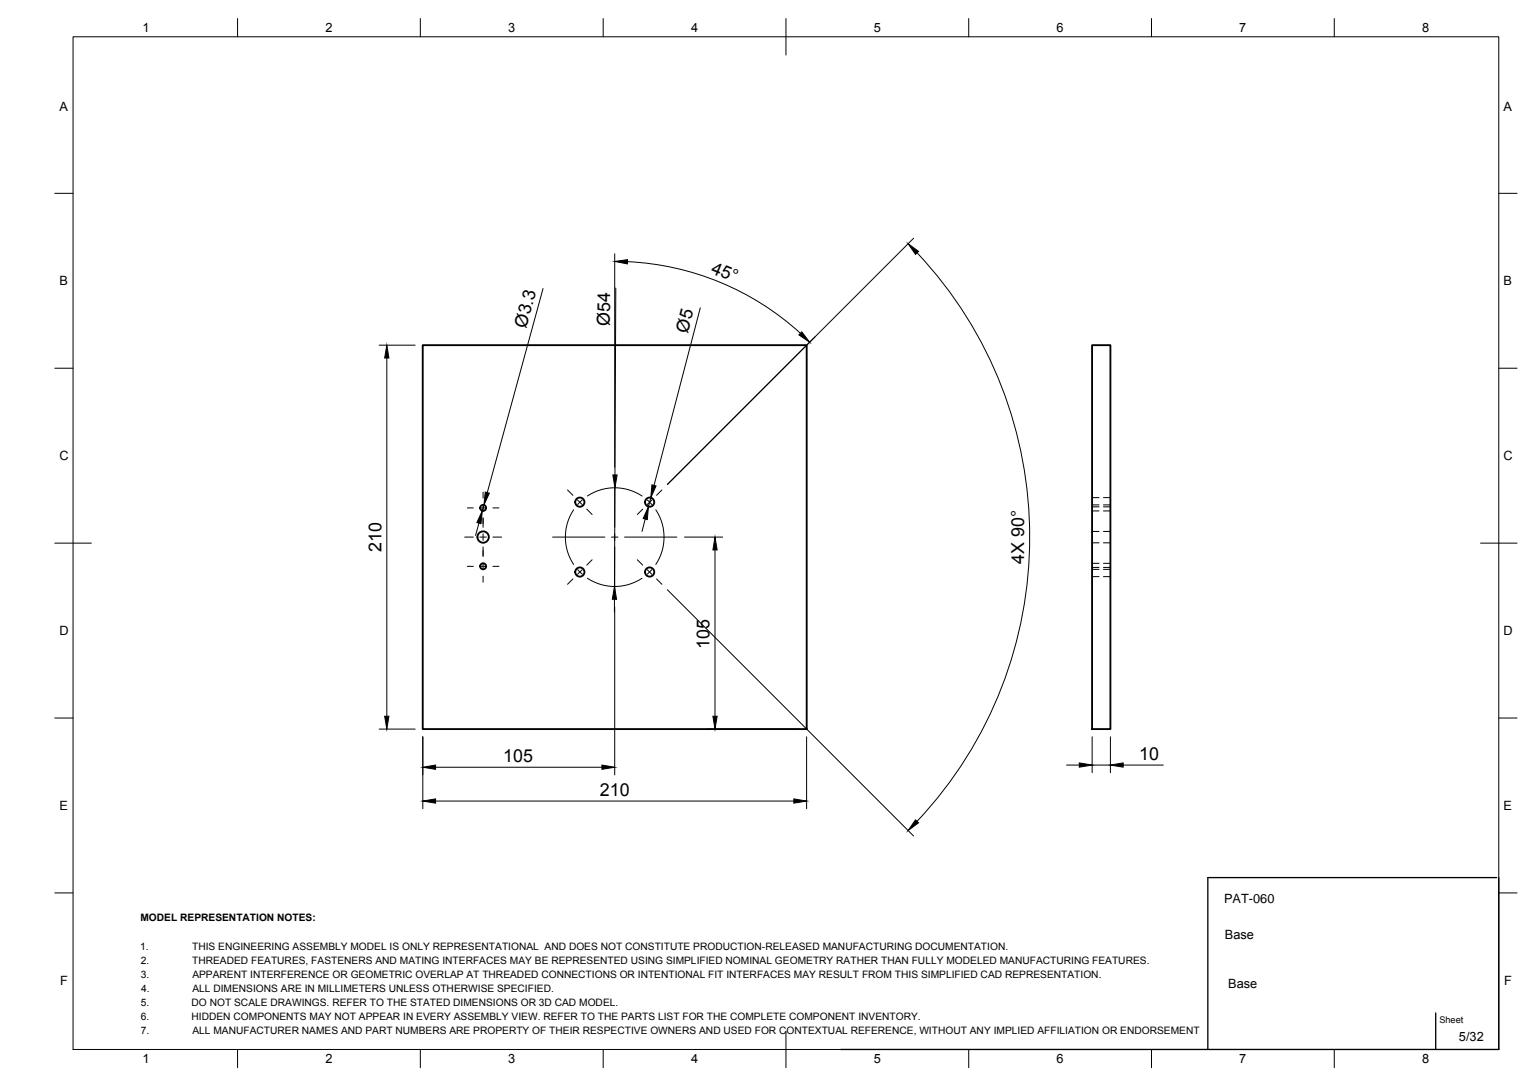
ISO-10303-21;
HEADER;
/* Generated by software containing ST-Developer
 * from STEP Tools, Inc. (www.steptools.com) 
 */

FILE_DESCRIPTION(
/* description */ ('Indexing fixture plate with plunger'),
/* implementation_level */ '2;1');

FILE_NAME(
/* name */ 'Base.step',
/* time_stamp */ '2026-10-28T03:23:41-07:00',
/* author */ (''),
/* organization */ (''),
/* preprocessor_version */ 'ST-DEVELOPER v20.2',
/* originating_system */ 'Autodesk Translation Framework v15.17.0.0',
/* authorisation */ '');

FILE_SCHEMA (('AUTOMOTIVE_DESIGN { 1 0 10303 214 3 1 1 }'));
ENDSEC;

DATA;
#10=MECHANICAL_DESIGN_GEOMETRIC_PRESENTATION_REPRESENTATION('',(#317),#10020);
#263=SHAPE_REPRESENTATION_RELATIONSHIP('SRR','None',#10137,#290);
#290=ADVANCED_BREP_SHAPE_REPRESENTATION('',(#353),#9990);
#317=STYLED_ITEM('',(#10347),#353);
#353=MANIFOLD_SOLID_BREP('Body1',#4571);
#387=FACE_BOUND('',#968,.T.);
#388=FACE_BOUND('',#969,.T.);
#389=FACE_BOUND('',#970,.T.);
#390=FACE_BOUND('',#971,.T.);
#391=FACE_BOUND('',#972,.T.);
#392=FACE_BOUND('',#973,.T.);
#393=FACE_BOUND('',#974,.T.);
#394=FACE_BOUND('',#976,.T.);
#395=FACE_BOUND('',#977,.T.);
#396=FACE_BOUND('',#978,.T.);
#397=FACE_BOUND('',#979,.T.);
#398=FACE_BOUND('',#980,.T.);
#399=FACE_BOUND('',#981,.T.);
#400=FACE_BOUND('',#982,.T.);
#537=PLANE('',#4931);
#538=PLANE('',#4932);
#539=PLANE('',#4933);
#540=PLANE('',#4934);
#541=PLANE('',#4935);
#542=PLANE('',#4936);
#670=FACE_OUTER_BOUND('',#956,.T.);
#671=FACE_OUTER_BOUND('',#957,.T.);
#672=FACE_OUTER_BOUND('',#958,.T.);
#673=FACE_OUTER_BOUND('',#959,.T.);
#674=FACE_OUTER_BOUND('',#960,.T.);
#675=FACE_OUTER_BOUND('',#961,.T.);
#676=FACE_OUTER_BOUND('',#962,.T.);
#677=FACE_OUTER_BOUND('',#963,.T.);
#678=FACE_OUTER_BOUND('',#964,.T.);
#679=FACE_OUTER_BOUND('',#965,.T.);
#680=FACE_OUTER_BOUND('',#966,.T.);
#681=FACE_OUTER_BOUND('',#967,.T.);
#682=FACE_OUTER_BOUND('',#975,.T.);
#956=EDGE_LOOP('',(#3063,#3064,#3065,#3066));
#957=EDGE_LOOP('',(#3067,#3068,#3069,#3070));
#958=EDGE_LOOP('',(#3071,#3072,#3073,#3074));
#959=EDGE_LOOP('',(#3075,#3076,#3077,#3078));
#960=EDGE_LOOP('',(#3079,#3080,#3081,#3082));
#961=EDGE_LOOP('',(#3083,#3084,#3085,#3086));
#962=EDGE_LOOP('',(#3087,#3088,#3089,#3090));
#963=EDGE_LOOP('',(#3091,#3092,#3093,#3094));
#964=EDGE_LOOP('',(#3095,#3096,#3097,#3098));
#965=EDGE_LOOP('',(#3099,#3100,#3101,#3102));
#966=EDGE_LOOP('',(#3103,#3104,#3105,#3106));
#967=EDGE_LOOP('',(#3107,#3108,#3109,#3110));
#968=EDGE_LOOP('',(#3111));
#969=EDGE_LOOP('',(#3112));
#970=EDGE_LOOP('',(#3113));
#971=EDGE_LOOP('',(#3114));
#972=EDGE_LOOP('',(#3115));
#973=EDGE_LOOP('',(#3116));
#974=EDGE_LOOP('',(#3117));
#975=EDGE_LOOP('',(#3118,#3119,#3120,#3121));
#976=EDGE_LOOP('',(#3122));
#977=EDGE_LOOP('',(#3123));
#978=EDGE_LOOP('',(#3124));
#979=EDGE_LOOP('',(#3125));
#980=EDGE_LOOP('',(#3126));
#981=EDGE_LOOP('',(#3127));
#982=EDGE_LOOP('',(#3128));
#1392=LINE('',#7132,#1612);
#1393=LINE('',#7138,#1613);
#1394=LINE('',#7144,#1614);
#1395=LINE('',#7150,#1615);
#1396=LINE('',#7156,#1616);
#1397=LINE('',#7162,#1617);
#1398=LINE('',#7168,#1618);
#1399=LINE('',#7173,#1619);
#1400=LINE('',#7175,#1620);
#1401=LINE('',#7177,#1621);
#1402=LINE('',#7178,#1622);
#1403=LINE('',#7181,#1623);
#1404=LINE('',#7183,#1624);
#1405=LINE('',#7184,#1625);
#1406=LINE('',#7187,#1626);
#1407=LINE('',#7189,#1627);
#1408=LINE('',#7190,#1628);
#1409=LINE('',#7192,#1629);
#1410=LINE('',#7193,#1630);
#1612=VECTOR('',#5583,0.165);
#1613=VECTOR('',#5590,0.165);
#1614=VECTOR('',#5597,0.31);
#1615=VECTOR('',#5604,0.25);
#1616=VECTOR('',#5611,0.25);
#1617=VECTOR('',#5618,0.25);
#1618=VECTOR('',#5625,0.25);
#1619=VECTOR('',#5630,1.);
#1620=VECTOR('',#5631,1.);
#1621=VECTOR('',#5632,1.);
#1622=VECTOR('',#5633,1.);
#1623=VECTOR('',#5636,1.);
#1624=VECTOR('',#5637,1.);
#1625=VECTOR('',#5638,1.);
#1626=VECTOR('',#5641,1.);
#1627=VECTOR('',#5642,1.);
#1628=VECTOR('',#5643,1.);
#1629=VECTOR('',#5646,1.);
#1630=VECTOR('',#5647,1.);
#1832=CIRCLE('',#4911,0.165);
#1833=CIRCLE('',#4912,0.165);
#1834=CIRCLE('',#4914,0.165);
#1835=CIRCLE('',#4915,0.165);
#1836=CIRCLE('',#4917,0.31);
#1837=CIRCLE('',#4918,0.31);
#1838=CIRCLE('',#4920,0.25);
#1839=CIRCLE('',#4921,0.25);
#1840=CIRCLE('',#4923,0.25);
#1841=CIRCLE('',#4924,0.25);
#1842=CIRCLE('',#4926,0.25);
#1843=CIRCLE('',#4927,0.25);
#1844=CIRCLE('',#4929,0.25);
#1845=CIRCLE('',#4930,0.25);
#2135=VERTEX_POINT('',#7129);
#2136=VERTEX_POINT('',#7131);
#2137=VERTEX_POINT('',#7135);
#2138=VERTEX_POINT('',#7137);
#2139=VERTEX_POINT('',#7141);
#2140=VERTEX_POINT('',#7143);
#2141=VERTEX_POINT('',#7147);
#2142=VERTEX_POINT('',#7149);
#2143=VERTEX_POINT('',#7153);
#2144=VERTEX_POINT('',#7155);
#2145=VERTEX_POINT('',#7159);
#2146=VERTEX_POINT('',#7161);
#2147=VERTEX_POINT('',#7165);
#2148=VERTEX_POINT('',#7167);
#2149=VERTEX_POINT('',#7171);
#2150=VERTEX_POINT('',#7172);
#2151=VERTEX_POINT('',#7174);
#2152=VERTEX_POINT('',#7176);
#2153=VERTEX_POINT('',#7180);
#2154=VERTEX_POINT('',#7182);
#2155=VERTEX_POINT('',#7186);
#2156=VERTEX_POINT('',#7188);
#2511=EDGE_CURVE('',#2135,#2135,#1832,.T.);
#2512=EDGE_CURVE('',#2135,#2136,#1392,.T.);
#2513=EDGE_CURVE('',#2136,#2136,#1833,.T.);
#2514=EDGE_CURVE('',#2137,#2137,#1834,.T.);
#2515=EDGE_CURVE('',#2137,#2138,#1393,.T.);
#2516=EDGE_CURVE('',#2138,#2138,#1835,.T.);
#2517=EDGE_CURVE('',#2139,#2139,#1836,.T.);
#2518=EDGE_CURVE('',#2139,#2140,#1394,.T.);
#2519=EDGE_CURVE('',#2140,#2140,#1837,.T.);
#2520=EDGE_CURVE('',#2141,#2141,#1838,.T.);
#2521=EDGE_CURVE('',#2141,#2142,#1395,.T.);
#2522=EDGE_CURVE('',#2142,#2142,#1839,.T.);
#2523=EDGE_CURVE('',#2143,#2143,#1840,.T.);
#2524=EDGE_CURVE('',#2143,#2144,#1396,.T.);
#2525=EDGE_CURVE('',#2144,#2144,#1841,.T.);
#2526=EDGE_CURVE('',#2145,#2145,#1842,.T.);
#2527=EDGE_CURVE('',#2145,#2146,#1397,.T.);
#2528=EDGE_CURVE('',#2146,#2146,#1843,.T.);
#2529=EDGE_CURVE('',#2147,#2147,#1844,.T.);
#2530=EDGE_CURVE('',#2147,#2148,#1398,.T.);
#2531=EDGE_CURVE('',#2148,#2148,#1845,.T.);
#2532=EDGE_CURVE('',#2149,#2150,#1399,.T.);
#2533=EDGE_CURVE('',#2150,#2151,#1400,.T.);
#2534=EDGE_CURVE('',#2152,#2151,#1401,.T.);
#2535=EDGE_CURVE('',#2149,#2152,#1402,.T.);
#2536=EDGE_CURVE('',#2153,#2149,#1403,.T.);
#2537=EDGE_CURVE('',#2154,#2152,#1404,.T.);
#2538=EDGE_CURVE('',#2153,#2154,#1405,.T.);
#2539=EDGE_CURVE('',#2155,#2153,#1406,.T.);
#2540=EDGE_CURVE('',#2156,#2154,#1407,.T.);
#2541=EDGE_CURVE('',#2155,#2156,#1408,.T.);
#2542=EDGE_CURVE('',#2150,#2155,#1409,.T.);
#2543=EDGE_CURVE('',#2151,#2156,#1410,.T.);
#3063=ORIENTED_EDGE('',*,*,#2511,.F.);
#3064=ORIENTED_EDGE('',*,*,#2512,.T.);
#3065=ORIENTED_EDGE('',*,*,#2513,.F.);
#3066=ORIENTED_EDGE('',*,*,#2512,.F.);
#3067=ORIENTED_EDGE('',*,*,#2514,.F.);
#3068=ORIENTED_EDGE('',*,*,#2515,.T.);
#3069=ORIENTED_EDGE('',*,*,#2516,.F.);
#3070=ORIENTED_EDGE('',*,*,#2515,.F.);
#3071=ORIENTED_EDGE('',*,*,#2517,.F.);
#3072=ORIENTED_EDGE('',*,*,#2518,.T.);
#3073=ORIENTED_EDGE('',*,*,#2519,.F.);
#3074=ORIENTED_EDGE('',*,*,#2518,.F.);
#3075=ORIENTED_EDGE('',*,*,#2520,.F.);
#3076=ORIENTED_EDGE('',*,*,#2521,.T.);
#3077=ORIENTED_EDGE('',*,*,#2522,.F.);
#3078=ORIENTED_EDGE('',*,*,#2521,.F.);
#3079=ORIENTED_EDGE('',*,*,#2523,.F.);
#3080=ORIENTED_EDGE('',*,*,#2524,.T.);
#3081=ORIENTED_EDGE('',*,*,#2525,.F.);
#3082=ORIENTED_EDGE('',*,*,#2524,.F.);
#3083=ORIENTED_EDGE('',*,*,#2526,.F.);
#3084=ORIENTED_EDGE('',*,*,#2527,.T.);
#3085=ORIENTED_EDGE('',*,*,#2528,.F.);
#3086=ORIENTED_EDGE('',*,*,#2527,.F.);
#3087=ORIENTED_EDGE('',*,*,#2529,.F.);
#3088=ORIENTED_EDGE('',*,*,#2530,.T.);
#3089=ORIENTED_EDGE('',*,*,#2531,.F.);
#3090=ORIENTED_EDGE('',*,*,#2530,.F.);
#3091=ORIENTED_EDGE('',*,*,#2532,.T.);
#3092=ORIENTED_EDGE('',*,*,#2533,.T.);
#3093=ORIENTED_EDGE('',*,*,#2534,.F.);
#3094=ORIENTED_EDGE('',*,*,#2535,.F.);
#3095=ORIENTED_EDGE('',*,*,#2536,.T.);
#3096=ORIENTED_EDGE('',*,*,#2535,.T.);
#3097=ORIENTED_EDGE('',*,*,#2537,.F.);
#3098=ORIENTED_EDGE('',*,*,#2538,.F.);
#3099=ORIENTED_EDGE('',*,*,#2539,.T.);
#3100=ORIENTED_EDGE('',*,*,#2538,.T.);
#3101=ORIENTED_EDGE('',*,*,#2540,.F.);
#3102=ORIENTED_EDGE('',*,*,#2541,.F.);
#3103=ORIENTED_EDGE('',*,*,#2542,.T.);
#3104=ORIENTED_EDGE('',*,*,#2541,.T.);
#3105=ORIENTED_EDGE('',*,*,#2543,.F.);
#3106=ORIENTED_EDGE('',*,*,#2533,.F.);
#3107=ORIENTED_EDGE('',*,*,#2543,.T.);
#3108=ORIENTED_EDGE('',*,*,#2540,.T.);
#3109=ORIENTED_EDGE('',*,*,#2537,.T.);
#3110=ORIENTED_EDGE('',*,*,#2534,.T.);
#3111=ORIENTED_EDGE('',*,*,#2531,.T.);
#3112=ORIENTED_EDGE('',*,*,#2528,.T.);
#3113=ORIENTED_EDGE('',*,*,#2525,.T.);
#3114=ORIENTED_EDGE('',*,*,#2522,.T.);
#3115=ORIENTED_EDGE('',*,*,#2519,.T.);
#3116=ORIENTED_EDGE('',*,*,#2516,.T.);
#3117=ORIENTED_EDGE('',*,*,#2513,.T.);
#3118=ORIENTED_EDGE('',*,*,#2542,.F.);
#3119=ORIENTED_EDGE('',*,*,#2532,.F.);
#3120=ORIENTED_EDGE('',*,*,#2536,.F.);
#3121=ORIENTED_EDGE('',*,*,#2539,.F.);
#3122=ORIENTED_EDGE('',*,*,#2529,.T.);
#3123=ORIENTED_EDGE('',*,*,#2526,.T.);
#3124=ORIENTED_EDGE('',*,*,#2523,.T.);
#3125=ORIENTED_EDGE('',*,*,#2520,.T.);
#3126=ORIENTED_EDGE('',*,*,#2517,.T.);
#3127=ORIENTED_EDGE('',*,*,#2514,.T.);
#3128=ORIENTED_EDGE('',*,*,#2511,.T.);
#4167=CYLINDRICAL_SURFACE('',#4910,0.165);
#4168=CYLINDRICAL_SURFACE('',#4913,0.165);
#4169=CYLINDRICAL_SURFACE('',#4916,0.31);
#4170=CYLINDRICAL_SURFACE('',#4919,0.25);
#4171=CYLINDRICAL_SURFACE('',#4922,0.25);
#4172=CYLINDRICAL_SURFACE('',#4925,0.25);
#4173=CYLINDRICAL_SURFACE('',#4928,0.25);
#4285=ADVANCED_FACE('',(#670),#4167,.F.);
#4286=ADVANCED_FACE('',(#671),#4168,.F.);
#4287=ADVANCED_FACE('',(#672),#4169,.F.);
#4288=ADVANCED_FACE('',(#673),#4170,.F.);
#4289=ADVANCED_FACE('',(#674),#4171,.F.);
#4290=ADVANCED_FACE('',(#675),#4172,.F.);
#4291=ADVANCED_FACE('',(#676),#4173,.F.);
#4292=ADVANCED_FACE('',(#677),#537,.T.);
#4293=ADVANCED_FACE('',(#678),#538,.T.);
#4294=ADVANCED_FACE('',(#679),#539,.T.);
#4295=ADVANCED_FACE('',(#680),#540,.T.);
#4296=ADVANCED_FACE('',(#681,#387,#388,#389,#390,#391,#392,#393),#541,.T.);
#4297=ADVANCED_FACE('',(#682,#394,#395,#396,#397,#398,#399,#400),#542,.F.);
#4571=CLOSED_SHELL('',(#4285,#4286,#4287,#4288,#4289,#4290,#4291,#4292,
#4293,#4294,#4295,#4296,#4297));
#4909=AXIS2_PLACEMENT_3D('',#7127,#5577,#5578);
#4910=AXIS2_PLACEMENT_3D('',#7128,#5579,#5580);
#4911=AXIS2_PLACEMENT_3D('',#7130,#5581,#5582);
#4912=AXIS2_PLACEMENT_3D('',#7133,#5584,#5585);
#4913=AXIS2_PLACEMENT_3D('',#7134,#5586,#5587);
#4914=AXIS2_PLACEMENT_3D('',#7136,#5588,#5589);
#4915=AXIS2_PLACEMENT_3D('',#7139,#5591,#5592);
#4916=AXIS2_PLACEMENT_3D('',#7140,#5593,#5594);
#4917=AXIS2_PLACEMENT_3D('',#7142,#5595,#5596);
#4918=AXIS2_PLACEMENT_3D('',#7145,#5598,#5599);
#4919=AXIS2_PLACEMENT_3D('',#7146,#5600,#5601);
#4920=AXIS2_PLACEMENT_3D('',#7148,#5602,#5603);
#4921=AXIS2_PLACEMENT_3D('',#7151,#5605,#5606);
#4922=AXIS2_PLACEMENT_3D('',#7152,#5607,#5608);
#4923=AXIS2_PLACEMENT_3D('',#7154,#5609,#5610);
#4924=AXIS2_PLACEMENT_3D('',#7157,#5612,#5613);
#4925=AXIS2_PLACEMENT_3D('',#7158,#5614,#5615);
#4926=AXIS2_PLACEMENT_3D('',#7160,#5616,#5617);
#4927=AXIS2_PLACEMENT_3D('',#7163,#5619,#5620);
#4928=AXIS2_PLACEMENT_3D('',#7164,#5621,#5622);
#4929=AXIS2_PLACEMENT_3D('',#7166,#5623,#5624);
#4930=AXIS2_PLACEMENT_3D('',#7169,#5626,#5627);
#4931=AXIS2_PLACEMENT_3D('',#7170,#5628,#5629);
#4932=AXIS2_PLACEMENT_3D('',#7179,#5634,#5635);
#4933=AXIS2_PLACEMENT_3D('',#7185,#5639,#5640);
#4934=AXIS2_PLACEMENT_3D('',#7191,#5644,#5645);
#4935=AXIS2_PLACEMENT_3D('',#7194,#5648,#5649);
#4936=AXIS2_PLACEMENT_3D('',#7195,#5650,#5651);
#5577=DIRECTION('axis',(0.,0.,1.));
#5578=DIRECTION('refdir',(1.,0.,0.));
#5579=DIRECTION('center_axis',(0.,0.,1.));
#5580=DIRECTION('ref_axis',(1.,0.,0.));
#5581=DIRECTION('center_axis',(0.,0.,1.));
#5582=DIRECTION('ref_axis',(1.,0.,0.));
#5583=DIRECTION('',(0.,0.,1.));
#5584=DIRECTION('center_axis',(0.,0.,-1.));
#5585=DIRECTION('ref_axis',(1.,0.,0.));
#5586=DIRECTION('center_axis',(0.,0.,1.));
#5587=DIRECTION('ref_axis',(1.,0.,0.));
#5588=DIRECTION('center_axis',(0.,0.,1.));
#5589=DIRECTION('ref_axis',(1.,0.,0.));
#5590=DIRECTION('',(0.,0.,1.));
#5591=DIRECTION('center_axis',(0.,0.,-1.));
#5592=DIRECTION('ref_axis',(1.,0.,0.));
#5593=DIRECTION('center_axis',(0.,0.,1.));
#5594=DIRECTION('ref_axis',(1.,0.,0.));
#5595=DIRECTION('center_axis',(0.,0.,1.));
#5596=DIRECTION('ref_axis',(1.,0.,0.));
#5597=DIRECTION('',(0.,0.,1.));
#5598=DIRECTION('center_axis',(0.,0.,-1.));
#5599=DIRECTION('ref_axis',(1.,0.,0.));
#5600=DIRECTION('center_axis',(0.,0.,1.));
#5601=DIRECTION('ref_axis',(1.,0.,0.));
#5602=DIRECTION('center_axis',(0.,0.,1.));
#5603=DIRECTION('ref_axis',(1.,0.,0.));
#5604=DIRECTION('',(0.,0.,1.));
#5605=DIRECTION('center_axis',(0.,0.,-1.));
#5606=DIRECTION('ref_axis',(1.,0.,0.));
#5607=DIRECTION('center_axis',(0.,0.,1.));
#5608=DIRECTION('ref_axis',(1.,0.,0.));
#5609=DIRECTION('center_axis',(0.,0.,1.));
#5610=DIRECTION('ref_axis',(1.,0.,0.));
#5611=DIRECTION('',(0.,0.,1.));
#5612=DIRECTION('center_axis',(0.,0.,-1.));
#5613=DIRECTION('ref_axis',(1.,0.,0.));
#5614=DIRECTION('center_axis',(0.,0.,1.));
#5615=DIRECTION('ref_axis',(1.,0.,0.));
#5616=DIRECTION('center_axis',(0.,0.,1.));
#5617=DIRECTION('ref_axis',(1.,0.,0.));
#5618=DIRECTION('',(0.,0.,1.));
#5619=DIRECTION('center_axis',(0.,0.,-1.));
#5620=DIRECTION('ref_axis',(1.,0.,0.));
#5621=DIRECTION('center_axis',(0.,0.,1.));
#5622=DIRECTION('ref_axis',(1.,0.,0.));
#5623=DIRECTION('center_axis',(0.,0.,1.));
#5624=DIRECTION('ref_axis',(1.,0.,0.));
#5625=DIRECTION('',(0.,0.,1.));
#5626=DIRECTION('center_axis',(0.,0.,-1.));
#5627=DIRECTION('ref_axis',(1.,0.,0.));
#5628=DIRECTION('center_axis',(0.,1.,0.));
#5629=DIRECTION('ref_axis',(-1.,0.,0.));
#5630=DIRECTION('',(-1.,0.,0.));
#5631=DIRECTION('',(0.,0.,1.));
#5632=DIRECTION('',(-1.,0.,0.));
#5633=DIRECTION('',(0.,0.,1.));
#5634=DIRECTION('center_axis',(1.,0.,0.));
#5635=DIRECTION('ref_axis',(0.,1.,0.));
#5636=DIRECTION('',(0.,1.,0.));
#5637=DIRECTION('',(0.,1.,0.));
#5638=DIRECTION('',(0.,0.,1.));
#5639=DIRECTION('center_axis',(0.,-1.,0.));
#5640=DIRECTION('ref_axis',(1.,0.,0.));
#5641=DIRECTION('',(1.,0.,0.));
#5642=DIRECTION('',(1.,0.,0.));
#5643=DIRECTION('',(0.,0.,1.));
#5644=DIRECTION('center_axis',(-1.,0.,0.));
#5645=DIRECTION('ref_axis',(0.,-1.,0.));
#5646=DIRECTION('',(0.,-1.,0.));
#5647=DIRECTION('',(0.,-1.,0.));
#5648=DIRECTION('center_axis',(0.,0.,1.));
#5649=DIRECTION('ref_axis',(1.,0.,0.));
#5650=DIRECTION('center_axis',(0.,0.,1.));
#5651=DIRECTION('ref_axis',(1.,0.,0.));
#7127=CARTESIAN_POINT('',(0.,0.,0.));
#7128=CARTESIAN_POINT('Origin',(7.2,1.6,-1.1));
#7129=CARTESIAN_POINT('',(7.035,1.6,-1.));
#7130=CARTESIAN_POINT('Origin',(7.2,1.6,-1.));
#7131=CARTESIAN_POINT('',(7.035,1.6,0.));
#7132=CARTESIAN_POINT('',(7.035,1.6,-1.1));
#7133=CARTESIAN_POINT('Origin',(7.2,1.6,0.));
#7134=CARTESIAN_POINT('Origin',(7.2,-1.6,-1.1));
#7135=CARTESIAN_POINT('',(7.035,-1.6,-1.));
#7136=CARTESIAN_POINT('Origin',(7.2,-1.6,-1.));
#7137=CARTESIAN_POINT('',(7.035,-1.6,0.));
#7138=CARTESIAN_POINT('',(7.035,-1.6,-1.1));
#7139=CARTESIAN_POINT('Origin',(7.2,-1.6,0.));
#7140=CARTESIAN_POINT('Origin',(7.2,0.,-1.1));
#7141=CARTESIAN_POINT('',(6.89,-3.79640507735679E-17,-1.));
#7142=CARTESIAN_POINT('Origin',(7.2,0.,-1.));
#7143=CARTESIAN_POINT('',(6.89,3.79640507735679E-17,0.));
#7144=CARTESIAN_POINT('',(6.89,-3.79640507735679E-17,-1.1));
#7145=CARTESIAN_POINT('Origin',(7.2,0.,0.));
#7146=CARTESIAN_POINT('Origin',(-1.90918830920368,-1.90918830920368,-1.1));
#7147=CARTESIAN_POINT('',(-2.15918830920368,-1.90918830920368,-1.));
#7148=CARTESIAN_POINT('Origin',(-1.90918830920368,-1.90918830920368,-1.));
#7149=CARTESIAN_POINT('',(-2.15918830920368,-1.90918830920368,0.));
#7150=CARTESIAN_POINT('',(-2.15918830920368,-1.90918830920368,-1.1));
#7151=CARTESIAN_POINT('Origin',(-1.90918830920368,-1.90918830920368,0.));
#7152=CARTESIAN_POINT('Origin',(-1.90918830920368,1.90918830920368,-1.1));
#7153=CARTESIAN_POINT('',(-2.15918830920368,1.90918830920368,-1.));
#7154=CARTESIAN_POINT('Origin',(-1.90918830920368,1.90918830920368,-1.));
#7155=CARTESIAN_POINT('',(-2.15918830920368,1.90918830920368,0.));
#7156=CARTESIAN_POINT('',(-2.15918830920368,1.90918830920368,-1.1));
#7157=CARTESIAN_POINT('Origin',(-1.90918830920368,1.90918830920368,0.));
#7158=CARTESIAN_POINT('Origin',(1.90918830920368,1.90918830920368,-1.1));
#7159=CARTESIAN_POINT('',(1.65918830920368,1.90918830920368,-1.));
#7160=CARTESIAN_POINT('Origin',(1.90918830920368,1.90918830920368,-1.));
#7161=CARTESIAN_POINT('',(1.65918830920368,1.90918830920368,0.));
#7162=CARTESIAN_POINT('',(1.65918830920368,1.90918830920368,-1.1));
#7163=CARTESIAN_POINT('Origin',(1.90918830920368,1.90918830920368,0.));
#7164=CARTESIAN_POINT('Origin',(1.90918830920368,-1.90918830920368,-1.1));
#7165=CARTESIAN_POINT('',(1.65918830920368,-1.90918830920368,-1.));
#7166=CARTESIAN_POINT('Origin',(1.90918830920368,-1.90918830920368,-1.));
#7167=CARTESIAN_POINT('',(1.65918830920368,-1.90918830920368,0.));
#7168=CARTESIAN_POINT('',(1.65918830920368,-1.90918830920368,-1.1));
#7169=CARTESIAN_POINT('Origin',(1.90918830920368,-1.90918830920368,0.));
#7170=CARTESIAN_POINT('Origin',(10.5,10.5,-1.));
#7171=CARTESIAN_POINT('',(10.5,10.5,-1.));
#7172=CARTESIAN_POINT('',(-10.5,10.5,-1.));
#7173=CARTESIAN_POINT('',(10.5,10.5,-1.));
#7174=CARTESIAN_POINT('',(-10.5,10.5,0.));
#7175=CARTESIAN_POINT('',(-10.5,10.5,-1.));
#7176=CARTESIAN_POINT('',(10.5,10.5,0.));
#7177=CARTESIAN_POINT('',(10.5,10.5,0.));
#7178=CARTESIAN_POINT('',(10.5,10.5,-1.));
#7179=CARTESIAN_POINT('Origin',(10.5,-10.5,-1.));
#7180=CARTESIAN_POINT('',(10.5,-10.5,-1.));
#7181=CARTESIAN_POINT('',(10.5,-10.5,-1.));
#7182=CARTESIAN_POINT('',(10.5,-10.5,0.));
#7183=CARTESIAN_POINT('',(10.5,-10.5,0.));
#7184=CARTESIAN_POINT('',(10.5,-10.5,-1.));
#7185=CARTESIAN_POINT('Origin',(-10.5,-10.5,-1.));
#7186=CARTESIAN_POINT('',(-10.5,-10.5,-1.));
#7187=CARTESIAN_POINT('',(-10.5,-10.5,-1.));
#7188=CARTESIAN_POINT('',(-10.5,-10.5,0.));
#7189=CARTESIAN_POINT('',(-10.5,-10.5,0.));
#7190=CARTESIAN_POINT('',(-10.5,-10.5,-1.));
#7191=CARTESIAN_POINT('Origin',(-10.5,10.5,-1.));
#7192=CARTESIAN_POINT('',(-10.5,10.5,-1.));
#7193=CARTESIAN_POINT('',(-10.5,10.5,0.));
#7194=CARTESIAN_POINT('Origin',(0.,0.,0.));
#7195=CARTESIAN_POINT('Origin',(0.,0.,-1.));
#9957=UNCERTAINTY_MEASURE_WITH_UNIT(LENGTH_MEASURE(0.001),#10021,
'DISTANCE_ACCURACY_VALUE',
'Maximum model space distance between geometric entities at asserted c
onnectivities');
#9987=UNCERTAINTY_MEASURE_WITH_UNIT(LENGTH_MEASURE(0.001),#10021,
'DISTANCE_ACCURACY_VALUE',
'Maximum model space distance between geometric entities at asserted c
onnectivities');
#9990=(
GEOMETRIC_REPRESENTATION_CONTEXT(3)
GLOBAL_UNCERTAINTY_ASSIGNED_CONTEXT((#9957))
GLOBAL_UNIT_ASSIGNED_CONTEXT((#10021,#10023,#10024))
REPRESENTATION_CONTEXT('','3D')
);
#10020=(
GEOMETRIC_REPRESENTATION_CONTEXT(3)
GLOBAL_UNCERTAINTY_ASSIGNED_CONTEXT((#9987))
GLOBAL_UNIT_ASSIGNED_CONTEXT((#10021,#10023,#10024))
REPRESENTATION_CONTEXT('','3D')
);
#10021=(
LENGTH_UNIT()
NAMED_UNIT(*)
SI_UNIT(.CENTI.,.METRE.)
);
#10023=(
NAMED_UNIT(*)
PLANE_ANGLE_UNIT()
SI_UNIT($,.RADIAN.)
);
#10024=(
NAMED_UNIT(*)
SI_UNIT($,.STERADIAN.)
SOLID_ANGLE_UNIT()
);
#10027=SHAPE_DEFINITION_REPRESENTATION(#10059,#10137);
#10059=PRODUCT_DEFINITION_SHAPE('',$,#10170);
#10137=SHAPE_REPRESENTATION('',(#4909),#9990);
#10167=PRODUCT_DEFINITION_CONTEXT('part definition',#10265,'design');
#10170=PRODUCT_DEFINITION('Base','Base',#10202,#10167);
#10202=PRODUCT_DEFINITION_FORMATION('',$,#10269);
#10265=APPLICATION_CONTEXT(
'Core Data for Automotive Mechanical Design Process');
#10266=PRODUCT_CONTEXT('part definition',#10265,'mechanical');
#10269=PRODUCT('Base','Base','Base',(#10266));
#10341=COLOUR_RGB('Dark Blue',0.08,0.2,0.34);
#10342=FILL_AREA_STYLE_COLOUR('',#10341);
#10343=FILL_AREA_STYLE('',(#10342));
#10344=SURFACE_STYLE_FILL_AREA(#10343);
#10345=SURFACE_SIDE_STYLE('',(#10344));
#10346=SURFACE_STYLE_USAGE(.BOTH.,#10345);
#10347=PRESENTATION_STYLE_ASSIGNMENT((#10346));
ENDSEC;
END-ISO-10303-21;
